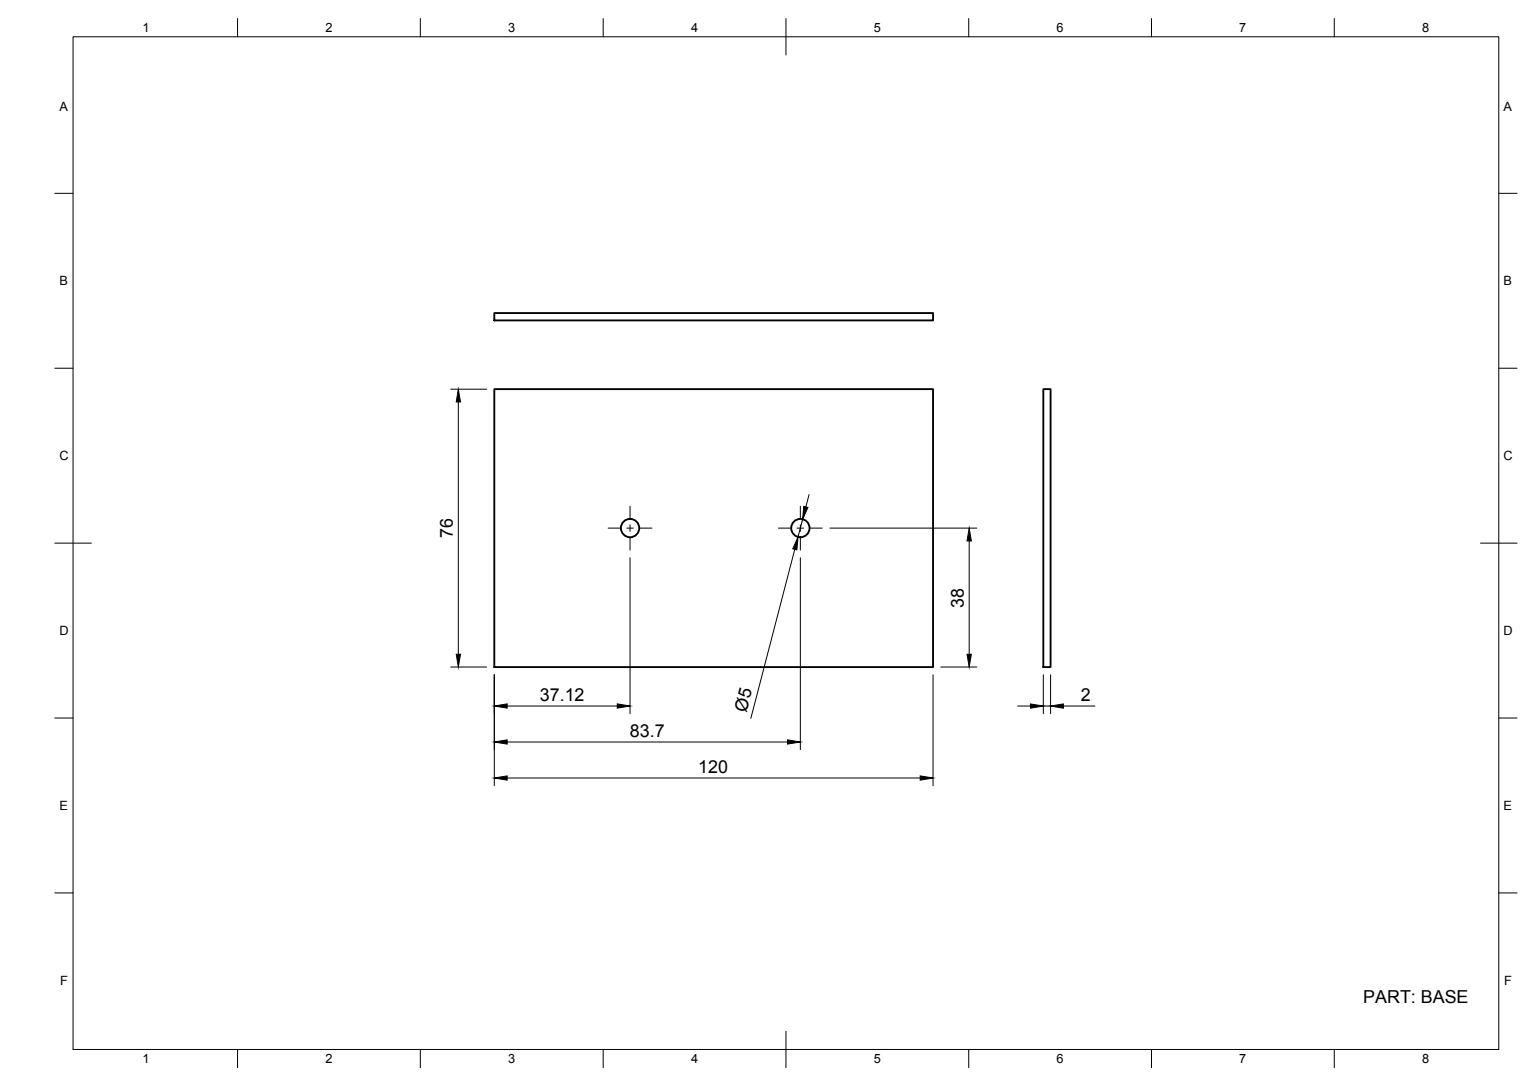
ISO-10303-21;
HEADER;
/* Generated by software containing ST-Developer
 * from STEP Tools, Inc. (www.steptools.com) 
 */

FILE_DESCRIPTION(
/* description */ (''),
/* implementation_level */ '2;1');

FILE_NAME(
/* name */ 'Base.step',
/* time_stamp */ '2026-09-20T21:52:48+06:00',
/* author */ (''),
/* organization */ (''),
/* preprocessor_version */ 'ST-DEVELOPER v20.2',
/* originating_system */ 'Autodesk Translation Framework v15.15.0.0',
/* authorisation */ '');

FILE_SCHEMA (('AUTOMOTIVE_DESIGN { 1 0 10303 214 3 1 1 }'));
ENDSEC;

DATA;
#10=MECHANICAL_DESIGN_GEOMETRIC_PRESENTATION_REPRESENTATION('',(#62),#2203);
#46=SHAPE_REPRESENTATION_RELATIONSHIP('SRR','None',#2238,#54);
#54=ADVANCED_BREP_SHAPE_REPRESENTATION('',(#70),#2198);
#62=STYLED_ITEM('',(#2286),#70);
#70=MANIFOLD_SOLID_BREP('Base',#1229);
#77=FACE_BOUND('',#268,.T.);
#78=FACE_BOUND('',#269,.T.);
#79=FACE_BOUND('',#275,.T.);
#80=FACE_BOUND('',#276,.T.);
#111=CIRCLE('',#1384,2.5);
#112=CIRCLE('',#1385,2.5);
#113=CIRCLE('',#1387,2.5);
#114=CIRCLE('',#1388,2.5);
#148=CYLINDRICAL_SURFACE('',#1383,2.5);
#149=CYLINDRICAL_SURFACE('',#1386,2.5);
#194=FACE_OUTER_BOUND('',#265,.T.);
#195=FACE_OUTER_BOUND('',#266,.T.);
#196=FACE_OUTER_BOUND('',#267,.T.);
#197=FACE_OUTER_BOUND('',#270,.T.);
#198=FACE_OUTER_BOUND('',#271,.T.);
#199=FACE_OUTER_BOUND('',#272,.T.);
#200=FACE_OUTER_BOUND('',#273,.T.);
#201=FACE_OUTER_BOUND('',#274,.T.);
#265=EDGE_LOOP('',(#958,#959,#960,#961));
#266=EDGE_LOOP('',(#962,#963,#964,#965));
#267=EDGE_LOOP('',(#966,#967,#968,#969));
#268=EDGE_LOOP('',(#970));
#269=EDGE_LOOP('',(#971));
#270=EDGE_LOOP('',(#972,#973,#974,#975));
#271=EDGE_LOOP('',(#976,#977,#978,#979));
#272=EDGE_LOOP('',(#980,#981,#982,#983));
#273=EDGE_LOOP('',(#984,#985,#986,#987));
#274=EDGE_LOOP('',(#988,#989,#990,#991));
#275=EDGE_LOOP('',(#992));
#276=EDGE_LOOP('',(#993));
#372=LINE('',#2012,#482);
#373=LINE('',#2018,#483);
#374=LINE('',#2023,#484);
#375=LINE('',#2025,#485);
#376=LINE('',#2027,#486);
#377=LINE('',#2028,#487);
#378=LINE('',#2031,#488);
#379=LINE('',#2033,#489);
#380=LINE('',#2034,#490);
#381=LINE('',#2037,#491);
#382=LINE('',#2038,#492);
#383=LINE('',#2041,#493);
#384=LINE('',#2042,#494);
#385=LINE('',#2044,#495);
#482=VECTOR('',#1640,2.5);
#483=VECTOR('',#1647,2.5);
#484=VECTOR('',#1652,10.);
#485=VECTOR('',#1653,10.);
#486=VECTOR('',#1654,10.);
#487=VECTOR('',#1655,10.);
#488=VECTOR('',#1658,10.);
#489=VECTOR('',#1659,10.);
#490=VECTOR('',#1660,10.);
#491=VECTOR('',#1663,10.);
#492=VECTOR('',#1664,10.);
#493=VECTOR('',#1667,10.);
#494=VECTOR('',#1668,10.);
#495=VECTOR('',#1671,10.);
#587=VERTEX_POINT('',#2009);
#588=VERTEX_POINT('',#2011);
#589=VERTEX_POINT('',#2015);
#590=VERTEX_POINT('',#2017);
#591=VERTEX_POINT('',#2021);
#592=VERTEX_POINT('',#2022);
#593=VERTEX_POINT('',#2024);
#594=VERTEX_POINT('',#2026);
#595=VERTEX_POINT('',#2030);
#596=VERTEX_POINT('',#2032);
#597=VERTEX_POINT('',#2036);
#598=VERTEX_POINT('',#2040);
#719=EDGE_CURVE('',#587,#587,#111,.T.);
#720=EDGE_CURVE('',#587,#588,#372,.T.);
#721=EDGE_CURVE('',#588,#588,#112,.T.);
#722=EDGE_CURVE('',#589,#589,#113,.T.);
#723=EDGE_CURVE('',#589,#590,#373,.T.);
#724=EDGE_CURVE('',#590,#590,#114,.T.);
#725=EDGE_CURVE('',#591,#592,#374,.T.);
#726=EDGE_CURVE('',#593,#591,#375,.T.);
#727=EDGE_CURVE('',#594,#593,#376,.T.);
#728=EDGE_CURVE('',#592,#594,#377,.T.);
#729=EDGE_CURVE('',#591,#595,#378,.T.);
#730=EDGE_CURVE('',#596,#595,#379,.T.);
#731=EDGE_CURVE('',#593,#596,#380,.T.);
#732=EDGE_CURVE('',#592,#597,#381,.T.);
#733=EDGE_CURVE('',#595,#597,#382,.T.);
#734=EDGE_CURVE('',#598,#596,#383,.T.);
#735=EDGE_CURVE('',#594,#598,#384,.T.);
#736=EDGE_CURVE('',#597,#598,#385,.T.);
#958=ORIENTED_EDGE('',*,*,#719,.F.);
#959=ORIENTED_EDGE('',*,*,#720,.T.);
#960=ORIENTED_EDGE('',*,*,#721,.F.);
#961=ORIENTED_EDGE('',*,*,#720,.F.);
#962=ORIENTED_EDGE('',*,*,#722,.F.);
#963=ORIENTED_EDGE('',*,*,#723,.T.);
#964=ORIENTED_EDGE('',*,*,#724,.T.);
#965=ORIENTED_EDGE('',*,*,#723,.F.);
#966=ORIENTED_EDGE('',*,*,#725,.F.);
#967=ORIENTED_EDGE('',*,*,#726,.F.);
#968=ORIENTED_EDGE('',*,*,#727,.F.);
#969=ORIENTED_EDGE('',*,*,#728,.F.);
#970=ORIENTED_EDGE('',*,*,#724,.F.);
#971=ORIENTED_EDGE('',*,*,#721,.T.);
#972=ORIENTED_EDGE('',*,*,#726,.T.);
#973=ORIENTED_EDGE('',*,*,#729,.T.);
#974=ORIENTED_EDGE('',*,*,#730,.F.);
#975=ORIENTED_EDGE('',*,*,#731,.F.);
#976=ORIENTED_EDGE('',*,*,#725,.T.);
#977=ORIENTED_EDGE('',*,*,#732,.T.);
#978=ORIENTED_EDGE('',*,*,#733,.F.);
#979=ORIENTED_EDGE('',*,*,#729,.F.);
#980=ORIENTED_EDGE('',*,*,#727,.T.);
#981=ORIENTED_EDGE('',*,*,#731,.T.);
#982=ORIENTED_EDGE('',*,*,#734,.F.);
#983=ORIENTED_EDGE('',*,*,#735,.F.);
#984=ORIENTED_EDGE('',*,*,#728,.T.);
#985=ORIENTED_EDGE('',*,*,#735,.T.);
#986=ORIENTED_EDGE('',*,*,#736,.F.);
#987=ORIENTED_EDGE('',*,*,#732,.F.);
#988=ORIENTED_EDGE('',*,*,#733,.T.);
#989=ORIENTED_EDGE('',*,*,#736,.T.);
#990=ORIENTED_EDGE('',*,*,#734,.T.);
#991=ORIENTED_EDGE('',*,*,#730,.T.);
#992=ORIENTED_EDGE('',*,*,#719,.T.);
#993=ORIENTED_EDGE('',*,*,#722,.T.);
#1134=PLANE('',#1389);
#1135=PLANE('',#1390);
#1136=PLANE('',#1391);
#1137=PLANE('',#1392);
#1138=PLANE('',#1393);
#1139=PLANE('',#1394);
#1190=ADVANCED_FACE('',(#194),#148,.F.);
#1191=ADVANCED_FACE('',(#195),#149,.F.);
#1192=ADVANCED_FACE('',(#196,#77,#78),#1134,.F.);
#1193=ADVANCED_FACE('',(#197),#1135,.T.);
#1194=ADVANCED_FACE('',(#198),#1136,.T.);
#1195=ADVANCED_FACE('',(#199),#1137,.T.);
#1196=ADVANCED_FACE('',(#200),#1138,.T.);
#1197=ADVANCED_FACE('',(#201,#79,#80),#1139,.T.);
#1229=CLOSED_SHELL('',(#1190,#1191,#1192,#1193,#1194,#1195,#1196,#1197));
#1382=AXIS2_PLACEMENT_3D('',#2007,#1634,#1635);
#1383=AXIS2_PLACEMENT_3D('',#2008,#1636,#1637);
#1384=AXIS2_PLACEMENT_3D('',#2010,#1638,#1639);
#1385=AXIS2_PLACEMENT_3D('',#2013,#1641,#1642);
#1386=AXIS2_PLACEMENT_3D('',#2014,#1643,#1644);
#1387=AXIS2_PLACEMENT_3D('',#2016,#1645,#1646);
#1388=AXIS2_PLACEMENT_3D('',#2019,#1648,#1649);
#1389=AXIS2_PLACEMENT_3D('',#2020,#1650,#1651);
#1390=AXIS2_PLACEMENT_3D('',#2029,#1656,#1657);
#1391=AXIS2_PLACEMENT_3D('',#2035,#1661,#1662);
#1392=AXIS2_PLACEMENT_3D('',#2039,#1665,#1666);
#1393=AXIS2_PLACEMENT_3D('',#2043,#1669,#1670);
#1394=AXIS2_PLACEMENT_3D('',#2045,#1672,#1673);
#1634=DIRECTION('axis',(0.,0.,1.));
#1635=DIRECTION('refdir',(1.,0.,0.));
#1636=DIRECTION('center_axis',(0.,-1.,0.));
#1637=DIRECTION('ref_axis',(1.,0.,0.));
#1638=DIRECTION('center_axis',(0.,-1.,0.));
#1639=DIRECTION('ref_axis',(1.,0.,0.));
#1640=DIRECTION('',(0.,-1.,0.));
#1641=DIRECTION('center_axis',(0.,1.,0.));
#1642=DIRECTION('ref_axis',(1.,0.,0.));
#1643=DIRECTION('center_axis',(0.,-1.,0.));
#1644=DIRECTION('ref_axis',(1.,0.,0.));
#1645=DIRECTION('center_axis',(0.,-1.,0.));
#1646=DIRECTION('ref_axis',(1.,0.,0.));
#1647=DIRECTION('',(0.,-1.,0.));
#1648=DIRECTION('center_axis',(0.,-1.,0.));
#1649=DIRECTION('ref_axis',(1.,0.,0.));
#1650=DIRECTION('center_axis',(0.,1.,0.));
#1651=DIRECTION('ref_axis',(0.,0.,1.));
#1652=DIRECTION('',(-1.,0.,0.));
#1653=DIRECTION('',(0.,0.,-1.));
#1654=DIRECTION('',(1.,0.,0.));
#1655=DIRECTION('',(0.,0.,1.));
#1656=DIRECTION('center_axis',(1.,0.,0.));
#1657=DIRECTION('ref_axis',(0.,0.,-1.));
#1658=DIRECTION('',(0.,1.,0.));
#1659=DIRECTION('',(0.,0.,-1.));
#1660=DIRECTION('',(0.,1.,0.));
#1661=DIRECTION('center_axis',(0.,0.,-1.));
#1662=DIRECTION('ref_axis',(-1.,0.,0.));
#1663=DIRECTION('',(0.,1.,0.));
#1664=DIRECTION('',(-1.,0.,0.));
#1665=DIRECTION('center_axis',(0.,0.,1.));
#1666=DIRECTION('ref_axis',(1.,0.,0.));
#1667=DIRECTION('',(1.,0.,0.));
#1668=DIRECTION('',(0.,1.,0.));
#1669=DIRECTION('center_axis',(-1.,0.,0.));
#1670=DIRECTION('ref_axis',(0.,0.,1.));
#1671=DIRECTION('',(0.,0.,1.));
#1672=DIRECTION('center_axis',(0.,1.,0.));
#1673=DIRECTION('ref_axis',(0.,0.,1.));
#2007=CARTESIAN_POINT('',(0.,0.,0.));
#2008=CARTESIAN_POINT('Origin',(0.,3.,26.3));
#2009=CARTESIAN_POINT('',(-2.5,5.,26.3));
#2010=CARTESIAN_POINT('Origin',(0.,5.,26.3));
#2011=CARTESIAN_POINT('',(-2.5,3.,26.3));
#2012=CARTESIAN_POINT('',(-2.5,3.,26.3));
#2013=CARTESIAN_POINT('Origin',(0.,3.,26.3));
#2014=CARTESIAN_POINT('Origin',(1.53080849893419E-15,3.,72.8759738016714));
#2015=CARTESIAN_POINT('',(-2.5,5.,72.8759738016714));
#2016=CARTESIAN_POINT('Origin',(1.53080849893419E-15,5.,72.8759738016714));
#2017=CARTESIAN_POINT('',(-2.5,3.,72.8759738016714));
#2018=CARTESIAN_POINT('',(-2.5,3.,72.8759738016714));
#2019=CARTESIAN_POINT('Origin',(1.53080849893419E-15,3.,72.8759738016714));
#2020=CARTESIAN_POINT('Origin',(0.,3.,50.));
#2021=CARTESIAN_POINT('',(38.,3.,-10.));
#2022=CARTESIAN_POINT('',(-38.,3.,-10.));
#2023=CARTESIAN_POINT('',(19.,3.,-10.));
#2024=CARTESIAN_POINT('',(38.,3.,110.));
#2025=CARTESIAN_POINT('',(38.,3.,80.));
#2026=CARTESIAN_POINT('',(-38.,3.,110.));
#2027=CARTESIAN_POINT('',(-19.,3.,110.));
#2028=CARTESIAN_POINT('',(-38.,3.,20.));
#2029=CARTESIAN_POINT('Origin',(38.,0.,110.));
#2030=CARTESIAN_POINT('',(38.,5.,-10.));
#2031=CARTESIAN_POINT('',(38.,0.,-10.));
#2032=CARTESIAN_POINT('',(38.,5.,110.));
#2033=CARTESIAN_POINT('',(38.,5.,-10.));
#2034=CARTESIAN_POINT('',(38.,0.,110.));
#2035=CARTESIAN_POINT('Origin',(38.,0.,-10.));
#2036=CARTESIAN_POINT('',(-38.,5.,-10.));
#2037=CARTESIAN_POINT('',(-38.,0.,-10.));
#2038=CARTESIAN_POINT('',(0.,5.,-10.));
#2039=CARTESIAN_POINT('Origin',(-38.,0.,110.));
#2040=CARTESIAN_POINT('',(-38.,5.,110.));
#2041=CARTESIAN_POINT('',(-38.,5.,110.));
#2042=CARTESIAN_POINT('',(-38.,0.,110.));
#2043=CARTESIAN_POINT('Origin',(-38.,0.,-10.));
#2044=CARTESIAN_POINT('',(-38.,5.,-10.));
#2045=CARTESIAN_POINT('Origin',(0.,5.,50.));
#2188=UNCERTAINTY_MEASURE_WITH_UNIT(LENGTH_MEASURE(0.01),#2204,
'DISTANCE_ACCURACY_VALUE',
'Maximum model space distance between geometric entities at asserted c
onnectivities');
#2193=UNCERTAINTY_MEASURE_WITH_UNIT(LENGTH_MEASURE(0.01),#2204,
'DISTANCE_ACCURACY_VALUE',
'Maximum model space distance between geometric entities at asserted c
onnectivities');
#2198=(
GEOMETRIC_REPRESENTATION_CONTEXT(3)
GLOBAL_UNCERTAINTY_ASSIGNED_CONTEXT((#2188))
GLOBAL_UNIT_ASSIGNED_CONTEXT((#2204,#2206,#2207))
REPRESENTATION_CONTEXT('','3D')
);
#2203=(
GEOMETRIC_REPRESENTATION_CONTEXT(3)
GLOBAL_UNCERTAINTY_ASSIGNED_CONTEXT((#2193))
GLOBAL_UNIT_ASSIGNED_CONTEXT((#2204,#2206,#2207))
REPRESENTATION_CONTEXT('','3D')
);
#2204=(
LENGTH_UNIT()
NAMED_UNIT(*)
SI_UNIT(.MILLI.,.METRE.)
);
#2206=(
NAMED_UNIT(*)
PLANE_ANGLE_UNIT()
SI_UNIT($,.RADIAN.)
);
#2207=(
NAMED_UNIT(*)
SI_UNIT($,.STERADIAN.)
SOLID_ANGLE_UNIT()
);
#2212=SHAPE_DEFINITION_REPRESENTATION(#2221,#2238);
#2221=PRODUCT_DEFINITION_SHAPE('',$,#2248);
#2238=SHAPE_REPRESENTATION('',(#1382),#2198);
#2243=PRODUCT_DEFINITION_CONTEXT('part definition',#2272,'design');
#2248=PRODUCT_DEFINITION('Base','Base',#2257,#2243);
#2257=PRODUCT_DEFINITION_FORMATION('',$,#2278);
#2272=APPLICATION_CONTEXT(
'Core Data for Automotive Mechanical Design Process');
#2273=PRODUCT_CONTEXT('part definition',#2272,'mechanical');
#2278=PRODUCT('Base','Base',$,(#2273));
#2286=PRESENTATION_STYLE_ASSIGNMENT((#2290));
#2290=SURFACE_STYLE_USAGE(.BOTH.,#2294);
#2294=SURFACE_SIDE_STYLE('',(#2298));
#2298=SURFACE_STYLE_FILL_AREA(#2302);
#2302=FILL_AREA_STYLE('Surface - Matte',(#2306));
#2306=FILL_AREA_STYLE_COLOUR('Surface - Matte',#2310);
#2310=COLOUR_RGB('Surface - Matte', 0.31764706, 0.68627451, 0.89019608);
ENDSEC;
END-ISO-10303-21;
